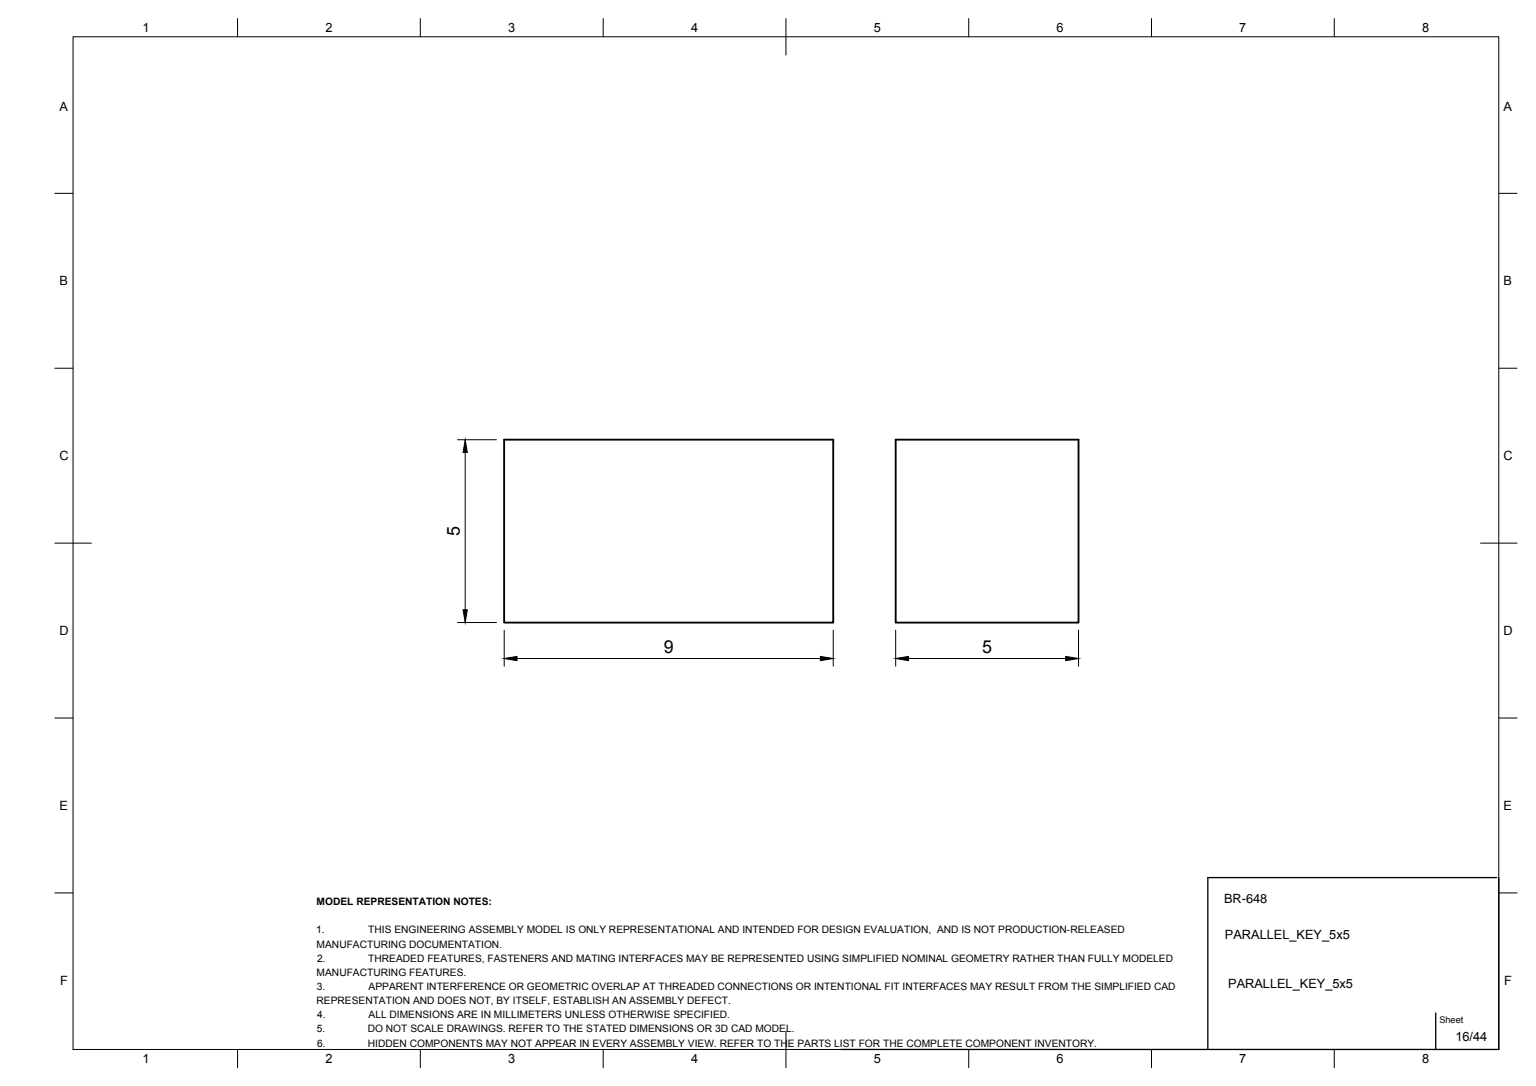
ISO-10303-21;
HEADER;
FILE_DESCRIPTION((''),'2;1');
FILE_NAME('PARALLEL_KEY_5x5.step','2026-10-01T22:05:39-07:00',(''),(''),'','','');
FILE_SCHEMA (('AUTOMOTIVE_DESIGN { 1 0 10303 214 3 1 1 }'));
ENDSEC;
DATA;
#10=MECHANICAL_DESIGN_GEOMETRIC_PRESENTATION_REPRESENTATION('',(#616),#24628);
#532=SHAPE_REPRESENTATION_RELATIONSHIP('SRR','None',#24804,#574) ;
#574=ADVANCED_BREP_SHAPE_REPRESENTATION('',(#656),#24594) ;
#616=STYLED_ITEM('',(#25030),#656) ;
#656=MANIFOLD_SOLID_BREP('PARALLEL_KEY_5x5',#13127) ;
#1291=LINE('',#21035,#2127) ;
#1292=LINE('',#21037,#2128) ;
#1293=LINE('',#21039,#2129) ;
#1294=LINE('',#21040,#2130) ;
#1295=LINE('',#21044,#2131) ;
#1296=LINE('',#21046,#2132) ;
#1297=LINE('',#21048,#2133) ;
#1298=LINE('',#21049,#2134) ;
#1299=LINE('',#21051,#2135) ;
#1300=LINE('',#21052,#2136) ;
#1301=LINE('',#21054,#2137) ;
#1302=LINE('',#21056,#2138) ;
#2127=VECTOR('',#16780,1.) ;
#2128=VECTOR('',#16781,1.) ;
#2129=VECTOR('',#16782,1.) ;
#2130=VECTOR('',#16783,1.) ;
#2131=VECTOR('',#16786,1.) ;
#2132=VECTOR('',#16787,1.) ;
#2133=VECTOR('',#16788,1.) ;
#2134=VECTOR('',#16789,1.) ;
#2135=VECTOR('',#16792,1.) ;
#2136=VECTOR('',#16793,1.) ;
#2137=VECTOR('',#16796,1.) ;
#2138=VECTOR('',#16799,1.) ;
#3206=FACE_OUTER_BOUND('',#4139,.T.) ;
#3207=FACE_OUTER_BOUND('',#4140,.T.) ;
#3208=FACE_OUTER_BOUND('',#4141,.T.) ;
#3209=FACE_OUTER_BOUND('',#4142,.T.) ;
#3210=FACE_OUTER_BOUND('',#4143,.T.) ;
#3211=FACE_OUTER_BOUND('',#4144,.T.) ;
#4139=EDGE_LOOP('',(#9639,#9640,#9641,#9642)) ;
#4140=EDGE_LOOP('',(#9643,#9644,#9645,#9646)) ;
#4141=EDGE_LOOP('',(#9647,#9648,#9649,#9650)) ;
#4142=EDGE_LOOP('',(#9651,#9652,#9653,#9654)) ;
#4143=EDGE_LOOP('',(#9655,#9656,#9657,#9658)) ;
#4144=EDGE_LOOP('',(#9659,#9660,#9661,#9662)) ;
#5921=VERTEX_POINT('',#21033) ;
#5922=VERTEX_POINT('',#21034) ;
#5923=VERTEX_POINT('',#21036) ;
#5924=VERTEX_POINT('',#21038) ;
#5925=VERTEX_POINT('',#21042) ;
#5926=VERTEX_POINT('',#21043) ;
#5927=VERTEX_POINT('',#21045) ;
#5928=VERTEX_POINT('',#21047) ;
#7309=EDGE_CURVE('',#5921,#5922,#1291,.T.) ;
#7310=EDGE_CURVE('',#5922,#5923,#1292,.T.) ;
#7311=EDGE_CURVE('',#5923,#5924,#1293,.T.) ;
#7312=EDGE_CURVE('',#5924,#5921,#1294,.T.) ;
#7313=EDGE_CURVE('',#5925,#5926,#1295,.T.) ;
#7314=EDGE_CURVE('',#5926,#5927,#1296,.T.) ;
#7315=EDGE_CURVE('',#5927,#5928,#1297,.T.) ;
#7316=EDGE_CURVE('',#5928,#5925,#1298,.T.) ;
#7317=EDGE_CURVE('',#5924,#5927,#1299,.T.) ;
#7318=EDGE_CURVE('',#5921,#5926,#1300,.T.) ;
#7319=EDGE_CURVE('',#5923,#5928,#1301,.T.) ;
#7320=EDGE_CURVE('',#5922,#5925,#1302,.T.) ;
#9639=ORIENTED_EDGE('',*,*,#7309,.T.) ;
#9640=ORIENTED_EDGE('',*,*,#7310,.T.) ;
#9641=ORIENTED_EDGE('',*,*,#7311,.T.) ;
#9642=ORIENTED_EDGE('',*,*,#7312,.T.) ;
#9643=ORIENTED_EDGE('',*,*,#7313,.T.) ;
#9644=ORIENTED_EDGE('',*,*,#7314,.T.) ;
#9645=ORIENTED_EDGE('',*,*,#7315,.T.) ;
#9646=ORIENTED_EDGE('',*,*,#7316,.T.) ;
#9647=ORIENTED_EDGE('',*,*,#7317,.T.) ;
#9648=ORIENTED_EDGE('',*,*,#7314,.F.) ;
#9649=ORIENTED_EDGE('',*,*,#7318,.F.) ;
#9650=ORIENTED_EDGE('',*,*,#7312,.F.) ;
#9651=ORIENTED_EDGE('',*,*,#7319,.T.) ;
#9652=ORIENTED_EDGE('',*,*,#7315,.F.) ;
#9653=ORIENTED_EDGE('',*,*,#7317,.F.) ;
#9654=ORIENTED_EDGE('',*,*,#7311,.F.) ;
#9655=ORIENTED_EDGE('',*,*,#7320,.T.) ;
#9656=ORIENTED_EDGE('',*,*,#7316,.F.) ;
#9657=ORIENTED_EDGE('',*,*,#7319,.F.) ;
#9658=ORIENTED_EDGE('',*,*,#7310,.F.) ;
#9659=ORIENTED_EDGE('',*,*,#7318,.T.) ;
#9660=ORIENTED_EDGE('',*,*,#7313,.F.) ;
#9661=ORIENTED_EDGE('',*,*,#7320,.F.) ;
#9662=ORIENTED_EDGE('',*,*,#7309,.F.) ;
#12118=PLANE('',#14201) ;
#12119=PLANE('',#14202) ;
#12120=PLANE('',#14203) ;
#12121=PLANE('',#14204) ;
#12122=PLANE('',#14205) ;
#12123=PLANE('',#14206) ;
#12601=ADVANCED_FACE('',(#3206),#12118,.T.) ;
#12602=ADVANCED_FACE('',(#3207),#12119,.F.) ;
#12603=ADVANCED_FACE('',(#3208),#12120,.F.) ;
#12604=ADVANCED_FACE('',(#3209),#12121,.F.) ;
#12605=ADVANCED_FACE('',(#3210),#12122,.F.) ;
#12606=ADVANCED_FACE('',(#3211),#12123,.F.) ;
#13127=CLOSED_SHELL('',(#12601,#12602,#12603,#12604,#12605,#12606)) ;
#14200=AXIS2_PLACEMENT_3D('',#21031,#16776,#16777) ;
#14201=AXIS2_PLACEMENT_3D('',#21032,#16778,#16779) ;
#14202=AXIS2_PLACEMENT_3D('',#21041,#16784,#16785) ;
#14203=AXIS2_PLACEMENT_3D('',#21050,#16790,#16791) ;
#14204=AXIS2_PLACEMENT_3D('',#21053,#16794,#16795) ;
#14205=AXIS2_PLACEMENT_3D('',#21055,#16797,#16798) ;
#14206=AXIS2_PLACEMENT_3D('',#21057,#16800,#16801) ;
#16776=DIRECTION('axis',(0.,0.,1.)) ;
#16777=DIRECTION('refdir',(1.,0.,0.)) ;
#16778=DIRECTION('center_axis',(0.,0.,1.)) ;
#16779=DIRECTION('ref_axis',(1.,0.,0.)) ;
#16780=DIRECTION('',(0.,1.,0.)) ;
#16781=DIRECTION('',(-1.,0.,0.)) ;
#16782=DIRECTION('',(0.,-1.,0.)) ;
#16783=DIRECTION('',(1.,0.,0.)) ;
#16784=DIRECTION('center_axis',(0.,0.,1.)) ;
#16785=DIRECTION('ref_axis',(1.,0.,0.)) ;
#16786=DIRECTION('',(0.,-1.,0.)) ;
#16787=DIRECTION('',(-1.,0.,0.)) ;
#16788=DIRECTION('',(0.,1.,0.)) ;
#16789=DIRECTION('',(1.,0.,0.)) ;
#16790=DIRECTION('center_axis',(0.,1.,0.)) ;
#16791=DIRECTION('ref_axis',(0.,0.,1.)) ;
#16792=DIRECTION('',(0.,0.,-1.)) ;
#16793=DIRECTION('',(0.,0.,-1.)) ;
#16794=DIRECTION('center_axis',(1.,0.,0.)) ;
#16795=DIRECTION('ref_axis',(0.,0.,-1.)) ;
#16796=DIRECTION('',(0.,0.,-1.)) ;
#16797=DIRECTION('center_axis',(0.,-1.,0.)) ;
#16798=DIRECTION('ref_axis',(0.,0.,-1.)) ;
#16799=DIRECTION('',(0.,0.,-1.)) ;
#16800=DIRECTION('center_axis',(-1.,0.,0.)) ;
#16801=DIRECTION('ref_axis',(0.,0.,1.)) ;
#21031=CARTESIAN_POINT('',(0.,0.,0.)) ;
#21032=CARTESIAN_POINT('Origin',(0.75,-6.15,0.25)) ;
#21033=CARTESIAN_POINT('',(1.,-6.6,0.25)) ;
#21034=CARTESIAN_POINT('',(1.,-5.7,0.25)) ;
#21035=CARTESIAN_POINT('',(1.,-6.15,0.25)) ;
#21036=CARTESIAN_POINT('',(0.5,-5.7,0.25)) ;
#21037=CARTESIAN_POINT('',(0.75,-5.7,0.25)) ;
#21038=CARTESIAN_POINT('',(0.5,-6.6,0.25)) ;
#21039=CARTESIAN_POINT('',(0.5,-6.15,0.25)) ;
#21040=CARTESIAN_POINT('',(0.75,-6.6,0.25)) ;
#21041=CARTESIAN_POINT('Origin',(0.75,-6.15,-0.25)) ;
#21042=CARTESIAN_POINT('',(1.,-5.7,-0.25)) ;
#21043=CARTESIAN_POINT('',(1.,-6.6,-0.25)) ;
#21044=CARTESIAN_POINT('',(1.,-6.15,-0.25)) ;
#21045=CARTESIAN_POINT('',(0.5,-6.6,-0.25)) ;
#21046=CARTESIAN_POINT('',(0.75,-6.6,-0.25)) ;
#21047=CARTESIAN_POINT('',(0.5,-5.7,-0.25)) ;
#21048=CARTESIAN_POINT('',(0.5,-6.15,-0.25)) ;
#21049=CARTESIAN_POINT('',(0.75,-5.7,-0.25)) ;
#21050=CARTESIAN_POINT('Origin',(0.75,-6.6,0.)) ;
#21051=CARTESIAN_POINT('',(0.5,-6.6,0.)) ;
#21052=CARTESIAN_POINT('',(1.,-6.6,0.)) ;
#21053=CARTESIAN_POINT('Origin',(0.5,-6.15,0.)) ;
#21054=CARTESIAN_POINT('',(0.5,-5.7,0.)) ;
#21055=CARTESIAN_POINT('Origin',(0.75,-5.7,0.)) ;
#21056=CARTESIAN_POINT('',(1.,-5.7,0.)) ;
#21057=CARTESIAN_POINT('Origin',(1.,-6.15,0.)) ;
#24546=UNCERTAINTY_MEASURE_WITH_UNIT(LENGTH_MEASURE(0.001),#24629,
'DISTANCE_ACCURACY_VALUE',
'Maximum model space distance between geometric entities at asserted c
onnectivities') ;
#24580=UNCERTAINTY_MEASURE_WITH_UNIT(LENGTH_MEASURE(0.001),#24629,
'DISTANCE_ACCURACY_VALUE',
'Maximum model space distance between geometric entities at asserted c
onnectivities') ;
#24594=(
GEOMETRIC_REPRESENTATION_CONTEXT(3)
GLOBAL_UNCERTAINTY_ASSIGNED_CONTEXT((#24546))
GLOBAL_UNIT_ASSIGNED_CONTEXT((#24629,#24631,#24632))
REPRESENTATION_CONTEXT('','3D')
) ;
#24628=(
GEOMETRIC_REPRESENTATION_CONTEXT(3)
GLOBAL_UNCERTAINTY_ASSIGNED_CONTEXT((#24580))
GLOBAL_UNIT_ASSIGNED_CONTEXT((#24629,#24631,#24632))
REPRESENTATION_CONTEXT('','3D')
) ;
#24629=(
LENGTH_UNIT()
NAMED_UNIT(*)
SI_UNIT(.CENTI.,.METRE.)
) ;
#24631=(
NAMED_UNIT(*)
PLANE_ANGLE_UNIT()
SI_UNIT($,.RADIAN.)
) ;
#24632=(
NAMED_UNIT(*)
SI_UNIT($,.STERADIAN.)
SOLID_ANGLE_UNIT()
) ;
#24646=SHAPE_DEFINITION_REPRESENTATION(#24693,#24804) ;
#24693=PRODUCT_DEFINITION_SHAPE('',$,#24852) ;
#24804=SHAPE_REPRESENTATION('',(#14200),#24594) ;
#24838=PRODUCT_DEFINITION_CONTEXT('part definition',#24981,'design') ;
#24852=PRODUCT_DEFINITION('PARALLEL_KEY_5x5','PARALLEL_KEY_5x5',
#24899,#24838) ;
#24899=PRODUCT_DEFINITION_FORMATION('',$,#24996) ;
#24981=APPLICATION_CONTEXT(
'Core Data for Automotive Mechanical Design Process') ;
#24982=PRODUCT_CONTEXT('part definition',#24981,'mechanical') ;
#24996=PRODUCT('PARALLEL_KEY_5x5','PARALLEL_KEY_5x5',$,(#24982)) ;
#25030=PRESENTATION_STYLE_ASSIGNMENT((#25040)) ;
#25040=SURFACE_STYLE_USAGE(.BOTH.,#25050) ;
#25050=SURFACE_SIDE_STYLE('',(#25060)) ;
#25060=SURFACE_STYLE_FILL_AREA(#25070) ;
#25070=FILL_AREA_STYLE('Steel - Satin',(#25080)) ;
#25080=FILL_AREA_STYLE_COLOUR('Steel - Satin',#25090) ;
#25090=COLOUR_RGB('Steel - Satin', 0.66274510, 0.83137255, 0.94901961) ;
ENDSEC;
END-ISO-10303-21;
